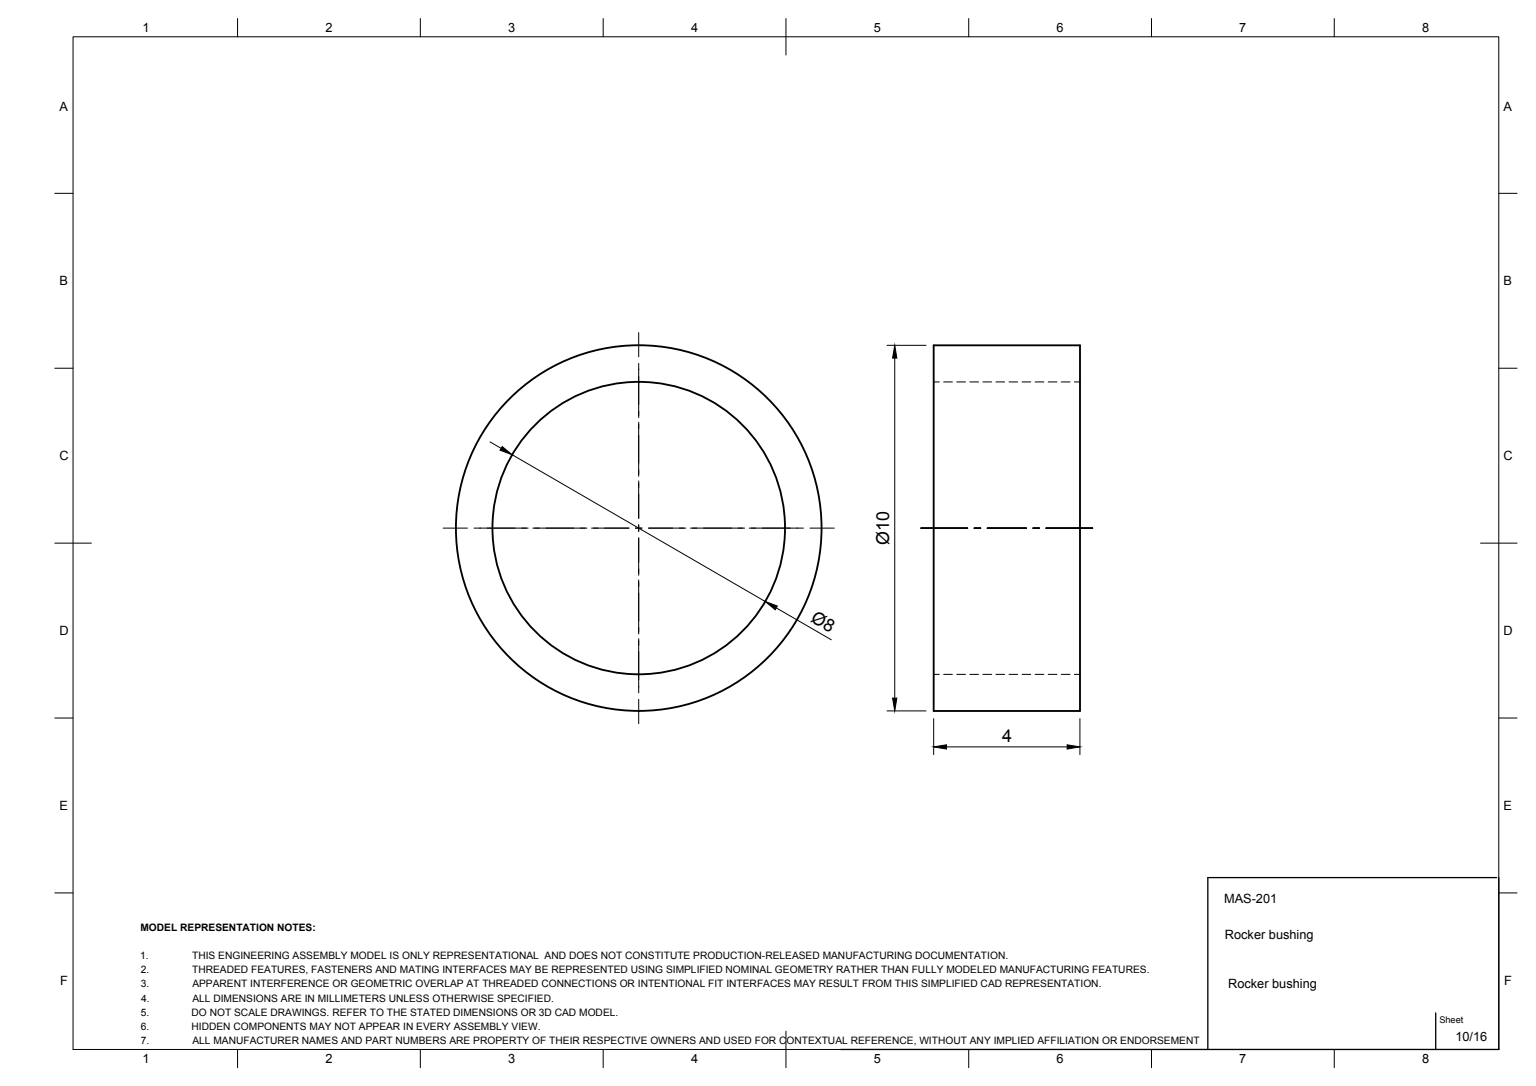
ISO-10303-21;
HEADER;
/* Generated by software containing ST-Developer
 * from STEP Tools, Inc. (www.steptools.com) 
 */

FILE_DESCRIPTION(
/* description */ ('Independent manual two-gate roller-track escapement for nominal30mm d
iameter20mm wide feed rollers. Opposed gates are driven by native capt
ured pin-slot loops with positive curved-slot travel stops at\X\B116de
g. Repeated gate/pin/washer/clip instances, adapted native common bear
ing families, full retaining lips and rotating polymer grip. External 
workpieces, gravity feeder/incline and mount anchors outside assembly.
 No powered-feed compatibility, impact, capacity, safety, force, wear 
or life rating.'),
/* implementation_level */ '2;1');

FILE_NAME(
/* name */ 'Rocker bushing.step',
/* time_stamp */ '2026-11-08T18:43:23-08:00',
/* author */ (''),
/* organization */ (''),
/* preprocessor_version */ 'ST-DEVELOPER v20.2',
/* originating_system */ 'Autodesk Translation Framework v15.17.0.0',
/* authorisation */ '');

FILE_SCHEMA (('AUTOMOTIVE_DESIGN { 1 0 10303 214 3 1 1 }'));
ENDSEC;

DATA;
#10=MECHANICAL_DESIGN_GEOMETRIC_PRESENTATION_REPRESENTATION('',(#463),#19863);
#425=SHAPE_REPRESENTATION_RELATIONSHIP('SRR','None',#19943,#444);
#444=ADVANCED_BREP_SHAPE_REPRESENTATION('',(#482),#19852);
#463=STYLED_ITEM('',(#20043),#482);
#482=MANIFOLD_SOLID_BREP('Body1',#6432);
#844=LINE('',#15875,#1309);
#845=LINE('',#15881,#1310);
#1309=VECTOR('',#8206,4.);
#1310=VECTOR('',#8213,5.);
#1548=CYLINDRICAL_SURFACE('',#6983,4.);
#1549=CYLINDRICAL_SURFACE('',#6986,5.);
#1667=FACE_BOUND('',#2337,.T.);
#1668=FACE_BOUND('',#2339,.T.);
#1925=FACE_OUTER_BOUND('',#2334,.T.);
#1926=FACE_OUTER_BOUND('',#2335,.T.);
#1927=FACE_OUTER_BOUND('',#2336,.T.);
#1928=FACE_OUTER_BOUND('',#2338,.T.);
#2334=EDGE_LOOP('',(#5373,#5374,#5375,#5376));
#2335=EDGE_LOOP('',(#5377,#5378,#5379,#5380));
#2336=EDGE_LOOP('',(#5381));
#2337=EDGE_LOOP('',(#5382));
#2338=EDGE_LOOP('',(#5383));
#2339=EDGE_LOOP('',(#5384));
#2562=CIRCLE('',#6984,4.);
#2563=CIRCLE('',#6985,4.);
#2564=CIRCLE('',#6987,5.);
#2565=CIRCLE('',#6988,5.);
#3036=VERTEX_POINT('',#15872);
#3037=VERTEX_POINT('',#15874);
#3038=VERTEX_POINT('',#15878);
#3039=VERTEX_POINT('',#15880);
#3845=EDGE_CURVE('',#3036,#3036,#2562,.T.);
#3846=EDGE_CURVE('',#3036,#3037,#844,.T.);
#3847=EDGE_CURVE('',#3037,#3037,#2563,.T.);
#3848=EDGE_CURVE('',#3038,#3038,#2564,.T.);
#3849=EDGE_CURVE('',#3038,#3039,#845,.T.);
#3850=EDGE_CURVE('',#3039,#3039,#2565,.T.);
#5373=ORIENTED_EDGE('',*,*,#3845,.F.);
#5374=ORIENTED_EDGE('',*,*,#3846,.T.);
#5375=ORIENTED_EDGE('',*,*,#3847,.T.);
#5376=ORIENTED_EDGE('',*,*,#3846,.F.);
#5377=ORIENTED_EDGE('',*,*,#3848,.F.);
#5378=ORIENTED_EDGE('',*,*,#3849,.T.);
#5379=ORIENTED_EDGE('',*,*,#3850,.T.);
#5380=ORIENTED_EDGE('',*,*,#3849,.F.);
#5381=ORIENTED_EDGE('',*,*,#3848,.T.);
#5382=ORIENTED_EDGE('',*,*,#3845,.T.);
#5383=ORIENTED_EDGE('',*,*,#3850,.F.);
#5384=ORIENTED_EDGE('',*,*,#3847,.F.);
#6020=PLANE('',#6989);
#6021=PLANE('',#6990);
#6304=ADVANCED_FACE('',(#1925),#1548,.F.);
#6305=ADVANCED_FACE('',(#1926),#1549,.T.);
#6306=ADVANCED_FACE('',(#1927,#1667),#6020,.T.);
#6307=ADVANCED_FACE('',(#1928,#1668),#6021,.F.);
#6432=CLOSED_SHELL('',(#6304,#6305,#6306,#6307));
#6982=AXIS2_PLACEMENT_3D('',#15870,#8200,#8201);
#6983=AXIS2_PLACEMENT_3D('',#15871,#8202,#8203);
#6984=AXIS2_PLACEMENT_3D('',#15873,#8204,#8205);
#6985=AXIS2_PLACEMENT_3D('',#15876,#8207,#8208);
#6986=AXIS2_PLACEMENT_3D('',#15877,#8209,#8210);
#6987=AXIS2_PLACEMENT_3D('',#15879,#8211,#8212);
#6988=AXIS2_PLACEMENT_3D('',#15882,#8214,#8215);
#6989=AXIS2_PLACEMENT_3D('',#15883,#8216,#8217);
#6990=AXIS2_PLACEMENT_3D('',#15884,#8218,#8219);
#8200=DIRECTION('axis',(0.,0.,1.));
#8201=DIRECTION('refdir',(1.,0.,0.));
#8202=DIRECTION('center_axis',(0.,0.,1.));
#8203=DIRECTION('ref_axis',(1.,0.,0.));
#8204=DIRECTION('center_axis',(0.,0.,-1.));
#8205=DIRECTION('ref_axis',(1.,0.,0.));
#8206=DIRECTION('',(0.,0.,-1.));
#8207=DIRECTION('center_axis',(0.,0.,-1.));
#8208=DIRECTION('ref_axis',(1.,0.,0.));
#8209=DIRECTION('center_axis',(0.,0.,1.));
#8210=DIRECTION('ref_axis',(1.,0.,0.));
#8211=DIRECTION('center_axis',(0.,0.,1.));
#8212=DIRECTION('ref_axis',(1.,0.,0.));
#8213=DIRECTION('',(0.,0.,-1.));
#8214=DIRECTION('center_axis',(0.,0.,1.));
#8215=DIRECTION('ref_axis',(1.,0.,0.));
#8216=DIRECTION('center_axis',(0.,0.,1.));
#8217=DIRECTION('ref_axis',(1.,0.,0.));
#8218=DIRECTION('center_axis',(0.,0.,1.));
#8219=DIRECTION('ref_axis',(1.,0.,0.));
#15870=CARTESIAN_POINT('',(0.,0.,0.));
#15871=CARTESIAN_POINT('Origin',(0.,0.,0.));
#15872=CARTESIAN_POINT('',(-4.,-4.89858719658941E-16,4.));
#15873=CARTESIAN_POINT('Origin',(0.,0.,4.));
#15874=CARTESIAN_POINT('',(-4.,-4.89858719658941E-16,0.));
#15875=CARTESIAN_POINT('',(-4.,-4.89858719658941E-16,0.));
#15876=CARTESIAN_POINT('Origin',(0.,0.,0.));
#15877=CARTESIAN_POINT('Origin',(0.,0.,0.));
#15878=CARTESIAN_POINT('',(-5.,-6.12323399573677E-16,4.));
#15879=CARTESIAN_POINT('Origin',(0.,0.,4.));
#15880=CARTESIAN_POINT('',(-5.,-6.12323399573677E-16,0.));
#15881=CARTESIAN_POINT('',(-5.,-6.12323399573677E-16,0.));
#15882=CARTESIAN_POINT('Origin',(0.,0.,0.));
#15883=CARTESIAN_POINT('Origin',(0.,0.,4.));
#15884=CARTESIAN_POINT('Origin',(0.,0.,0.));
#19831=UNCERTAINTY_MEASURE_WITH_UNIT(LENGTH_MEASURE(0.01),#19864,
'DISTANCE_ACCURACY_VALUE',
'Maximum model space distance between geometric entities at asserted c
onnectivities');
#19842=UNCERTAINTY_MEASURE_WITH_UNIT(LENGTH_MEASURE(0.01),#19864,
'DISTANCE_ACCURACY_VALUE',
'Maximum model space distance between geometric entities at asserted c
onnectivities');
#19852=(
GEOMETRIC_REPRESENTATION_CONTEXT(3)
GLOBAL_UNCERTAINTY_ASSIGNED_CONTEXT((#19831))
GLOBAL_UNIT_ASSIGNED_CONTEXT((#19864,#19866,#19867))
REPRESENTATION_CONTEXT('','3D')
);
#19863=(
GEOMETRIC_REPRESENTATION_CONTEXT(3)
GLOBAL_UNCERTAINTY_ASSIGNED_CONTEXT((#19842))
GLOBAL_UNIT_ASSIGNED_CONTEXT((#19864,#19866,#19867))
REPRESENTATION_CONTEXT('','3D')
);
#19864=(
LENGTH_UNIT()
NAMED_UNIT(*)
SI_UNIT(.MILLI.,.METRE.)
);
#19866=(
NAMED_UNIT(*)
PLANE_ANGLE_UNIT()
SI_UNIT($,.RADIAN.)
);
#19867=(
NAMED_UNIT(*)
SI_UNIT($,.STERADIAN.)
SOLID_ANGLE_UNIT()
);
#19877=SHAPE_DEFINITION_REPRESENTATION(#19897,#19943);
#19897=PRODUCT_DEFINITION_SHAPE('',$,#19964);
#19943=SHAPE_REPRESENTATION('',(#6982),#19852);
#19954=PRODUCT_DEFINITION_CONTEXT('part definition',#20016,'design');
#19964=PRODUCT_DEFINITION('Rocker bushing','Rocker bushing',#19984,#19954);
#19984=PRODUCT_DEFINITION_FORMATION('',$,#20027);
#20016=APPLICATION_CONTEXT(
'Core Data for Automotive Mechanical Design Process');
#20017=PRODUCT_CONTEXT('part definition',#20016,'mechanical');
#20027=PRODUCT('Rocker bushing','Rocker bushing',$,(#20017));
#20043=PRESENTATION_STYLE_ASSIGNMENT((#20050));
#20050=SURFACE_STYLE_USAGE(.BOTH.,#20057);
#20057=SURFACE_SIDE_STYLE('',(#20064));
#20064=SURFACE_STYLE_FILL_AREA(#20071);
#20071=FILL_AREA_STYLE('Light gray',(#20078));
#20078=FILL_AREA_STYLE_COLOUR('Light gray',#20085);
#20085=COLOUR_RGB('Light gray',0.725490196078431,0.752941176470588,0.792156862745098);
ENDSEC;
END-ISO-10303-21;
